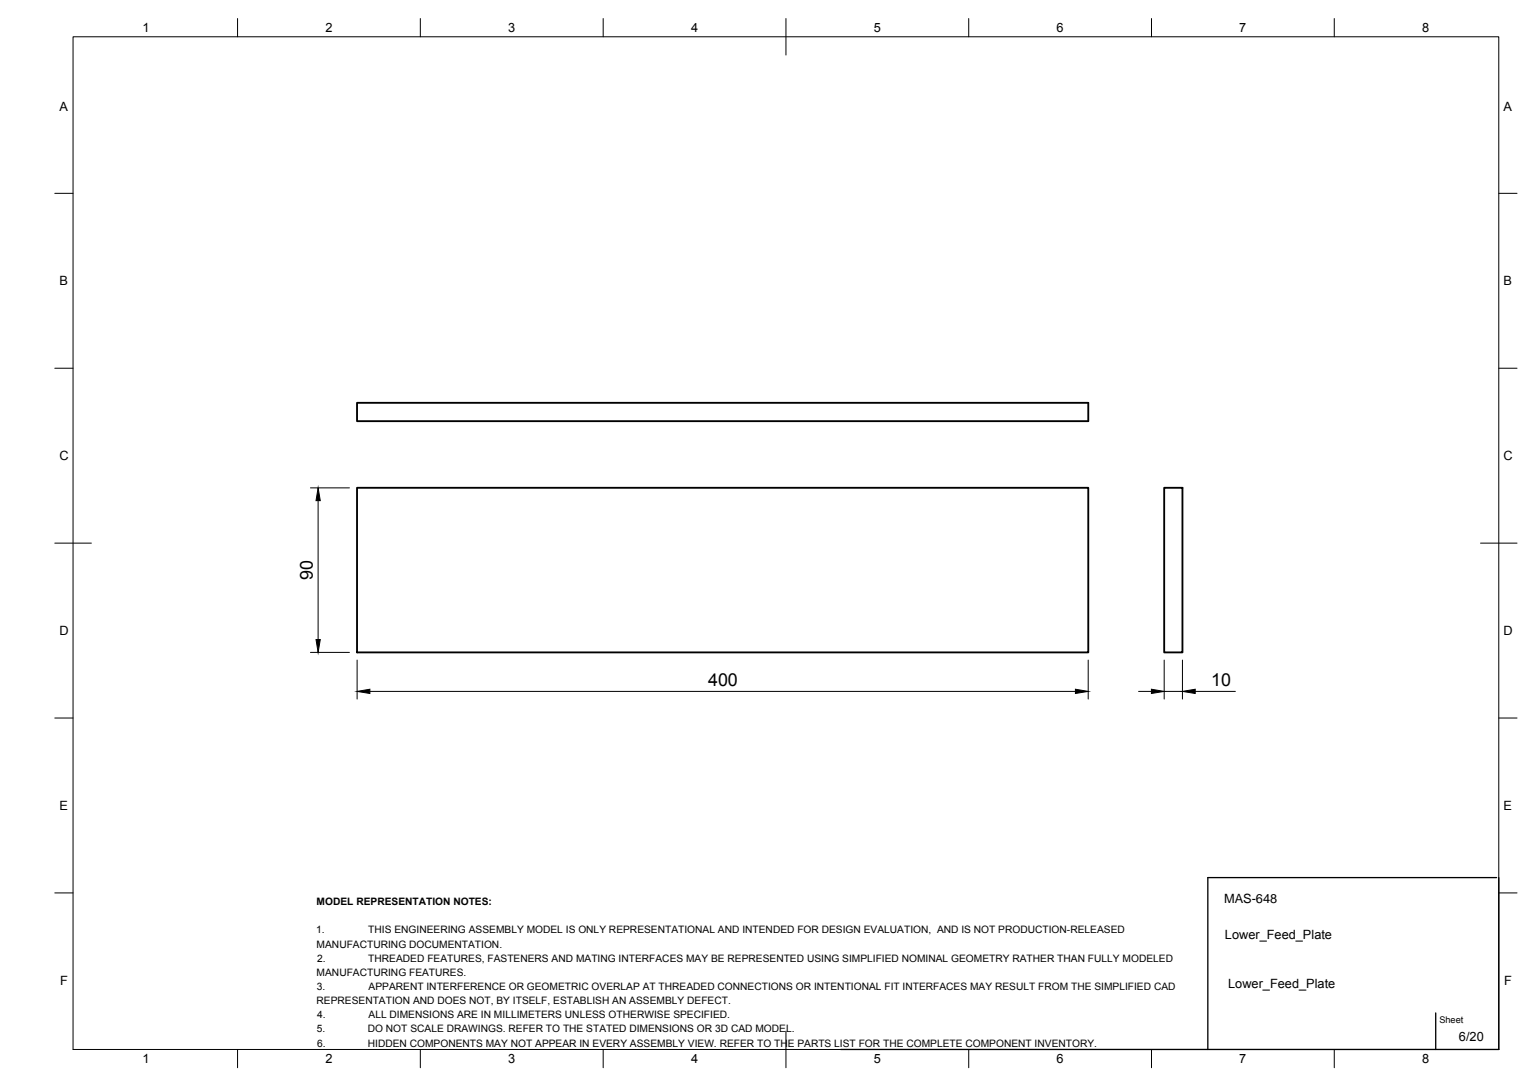
ISO-10303-21;
HEADER;
FILE_DESCRIPTION((''),'2;1');
FILE_NAME('Lower_Feed_Plate.step','2026-10-09T12:47:58-07:00',(''),(''),'','','');
FILE_SCHEMA (('AUTOMOTIVE_DESIGN { 1 0 10303 214 3 1 1 }'));
ENDSEC;
DATA;
#10=MECHANICAL_DESIGN_GEOMETRIC_PRESENTATION_REPRESENTATION('',(#310),#3475);
#286=SHAPE_REPRESENTATION_RELATIONSHIP('SRR','None',#3540,#298) ;
#298=ADVANCED_BREP_SHAPE_REPRESENTATION('',(#322),#3460) ;
#310=STYLED_ITEM('',(#3628),#322) ;
#322=MANIFOLD_SOLID_BREP('Body1',#1824) ;
#334=FACE_OUTER_BOUND('',#448,.T.) ;
#335=FACE_OUTER_BOUND('',#449,.T.) ;
#336=FACE_OUTER_BOUND('',#450,.T.) ;
#337=FACE_OUTER_BOUND('',#451,.T.) ;
#338=FACE_OUTER_BOUND('',#452,.T.) ;
#339=FACE_OUTER_BOUND('',#453,.T.) ;
#448=EDGE_LOOP('',(#1194,#1195,#1196,#1197)) ;
#449=EDGE_LOOP('',(#1198,#1199,#1200,#1201)) ;
#450=EDGE_LOOP('',(#1202,#1203,#1204,#1205)) ;
#451=EDGE_LOOP('',(#1206,#1207,#1208,#1209)) ;
#452=EDGE_LOOP('',(#1210,#1211,#1212,#1213)) ;
#453=EDGE_LOOP('',(#1214,#1215,#1216,#1217)) ;
#587=LINE('',#2829,#706) ;
#588=LINE('',#2831,#707) ;
#589=LINE('',#2833,#708) ;
#590=LINE('',#2834,#709) ;
#591=LINE('',#2837,#710) ;
#592=LINE('',#2839,#711) ;
#593=LINE('',#2840,#712) ;
#594=LINE('',#2843,#713) ;
#595=LINE('',#2845,#714) ;
#596=LINE('',#2846,#715) ;
#597=LINE('',#2848,#716) ;
#598=LINE('',#2849,#717) ;
#706=VECTOR('',#2222,1000.) ;
#707=VECTOR('',#2223,1000.) ;
#708=VECTOR('',#2224,1000.) ;
#709=VECTOR('',#2225,1000.) ;
#710=VECTOR('',#2228,1000.) ;
#711=VECTOR('',#2229,1000.) ;
#712=VECTOR('',#2230,1000.) ;
#713=VECTOR('',#2233,1000.) ;
#714=VECTOR('',#2234,1000.) ;
#715=VECTOR('',#2235,1000.) ;
#716=VECTOR('',#2238,1000.) ;
#717=VECTOR('',#2239,1000.) ;
#825=VERTEX_POINT('',#2827) ;
#826=VERTEX_POINT('',#2828) ;
#827=VERTEX_POINT('',#2830) ;
#828=VERTEX_POINT('',#2832) ;
#829=VERTEX_POINT('',#2836) ;
#830=VERTEX_POINT('',#2838) ;
#831=VERTEX_POINT('',#2842) ;
#832=VERTEX_POINT('',#2844) ;
#969=EDGE_CURVE('',#825,#826,#587,.T.) ;
#970=EDGE_CURVE('',#827,#825,#588,.T.) ;
#971=EDGE_CURVE('',#827,#828,#589,.T.) ;
#972=EDGE_CURVE('',#828,#826,#590,.T.) ;
#973=EDGE_CURVE('',#829,#825,#591,.T.) ;
#974=EDGE_CURVE('',#830,#829,#592,.T.) ;
#975=EDGE_CURVE('',#830,#827,#593,.T.) ;
#976=EDGE_CURVE('',#831,#829,#594,.T.) ;
#977=EDGE_CURVE('',#832,#831,#595,.T.) ;
#978=EDGE_CURVE('',#832,#830,#596,.T.) ;
#979=EDGE_CURVE('',#826,#831,#597,.T.) ;
#980=EDGE_CURVE('',#828,#832,#598,.T.) ;
#1194=ORIENTED_EDGE('',*,*,#969,.F.) ;
#1195=ORIENTED_EDGE('',*,*,#970,.F.) ;
#1196=ORIENTED_EDGE('',*,*,#971,.T.) ;
#1197=ORIENTED_EDGE('',*,*,#972,.T.) ;
#1198=ORIENTED_EDGE('',*,*,#973,.F.) ;
#1199=ORIENTED_EDGE('',*,*,#974,.F.) ;
#1200=ORIENTED_EDGE('',*,*,#975,.T.) ;
#1201=ORIENTED_EDGE('',*,*,#970,.T.) ;
#1202=ORIENTED_EDGE('',*,*,#976,.F.) ;
#1203=ORIENTED_EDGE('',*,*,#977,.F.) ;
#1204=ORIENTED_EDGE('',*,*,#978,.T.) ;
#1205=ORIENTED_EDGE('',*,*,#974,.T.) ;
#1206=ORIENTED_EDGE('',*,*,#979,.F.) ;
#1207=ORIENTED_EDGE('',*,*,#972,.F.) ;
#1208=ORIENTED_EDGE('',*,*,#980,.T.) ;
#1209=ORIENTED_EDGE('',*,*,#977,.T.) ;
#1210=ORIENTED_EDGE('',*,*,#971,.F.) ;
#1211=ORIENTED_EDGE('',*,*,#975,.F.) ;
#1212=ORIENTED_EDGE('',*,*,#978,.F.) ;
#1213=ORIENTED_EDGE('',*,*,#980,.F.) ;
#1214=ORIENTED_EDGE('',*,*,#969,.T.) ;
#1215=ORIENTED_EDGE('',*,*,#979,.T.) ;
#1216=ORIENTED_EDGE('',*,*,#976,.T.) ;
#1217=ORIENTED_EDGE('',*,*,#973,.T.) ;
#1644=PLANE('',#1972) ;
#1645=PLANE('',#1973) ;
#1646=PLANE('',#1974) ;
#1647=PLANE('',#1975) ;
#1648=PLANE('',#1976) ;
#1649=PLANE('',#1977) ;
#1710=ADVANCED_FACE('',(#334),#1644,.T.) ;
#1711=ADVANCED_FACE('',(#335),#1645,.T.) ;
#1712=ADVANCED_FACE('',(#336),#1646,.T.) ;
#1713=ADVANCED_FACE('',(#337),#1647,.T.) ;
#1714=ADVANCED_FACE('',(#338),#1648,.F.) ;
#1715=ADVANCED_FACE('',(#339),#1649,.T.) ;
#1824=CLOSED_SHELL('',(#1710,#1711,#1712,#1713,#1714,#1715)) ;
#1971=AXIS2_PLACEMENT_3D('',#2825,#2218,#2219) ;
#1972=AXIS2_PLACEMENT_3D('',#2826,#2220,#2221) ;
#1973=AXIS2_PLACEMENT_3D('',#2835,#2226,#2227) ;
#1974=AXIS2_PLACEMENT_3D('',#2841,#2231,#2232) ;
#1975=AXIS2_PLACEMENT_3D('',#2847,#2236,#2237) ;
#1976=AXIS2_PLACEMENT_3D('',#2850,#2240,#2241) ;
#1977=AXIS2_PLACEMENT_3D('',#2851,#2242,#2243) ;
#2218=DIRECTION('axis',(0.,0.,1.)) ;
#2219=DIRECTION('refdir',(1.,0.,0.)) ;
#2220=DIRECTION('center_axis',(-1.,0.,0.)) ;
#2221=DIRECTION('ref_axis',(0.,0.,1.)) ;
#2222=DIRECTION('',(0.,-1.,0.)) ;
#2223=DIRECTION('',(0.,0.,1.)) ;
#2224=DIRECTION('',(0.,-1.,0.)) ;
#2225=DIRECTION('',(0.,0.,1.)) ;
#2226=DIRECTION('center_axis',(-1.21430643318376E-16,1.,0.)) ;
#2227=DIRECTION('ref_axis',(-1.,-1.21430643318376E-16,0.)) ;
#2228=DIRECTION('',(-1.,-1.21430643318376E-16,0.)) ;
#2229=DIRECTION('',(0.,0.,1.)) ;
#2230=DIRECTION('',(-1.,-1.21430643318376E-16,0.)) ;
#2231=DIRECTION('center_axis',(1.,0.,0.)) ;
#2232=DIRECTION('ref_axis',(0.,0.,-1.)) ;
#2233=DIRECTION('',(0.,1.,0.)) ;
#2234=DIRECTION('',(0.,0.,1.)) ;
#2235=DIRECTION('',(0.,1.,0.)) ;
#2236=DIRECTION('center_axis',(1.21430643318376E-16,-1.,0.)) ;
#2237=DIRECTION('ref_axis',(1.,1.21430643318376E-16,0.)) ;
#2238=DIRECTION('',(1.,1.21430643318376E-16,0.)) ;
#2239=DIRECTION('',(1.,1.21430643318376E-16,0.)) ;
#2240=DIRECTION('center_axis',(0.,0.,1.)) ;
#2241=DIRECTION('ref_axis',(1.,0.,0.)) ;
#2242=DIRECTION('center_axis',(0.,0.,1.)) ;
#2243=DIRECTION('ref_axis',(1.,0.,0.)) ;
#2825=CARTESIAN_POINT('',(0.,0.,0.)) ;
#2826=CARTESIAN_POINT('Origin',(-200.,-45.,-10.)) ;
#2827=CARTESIAN_POINT('',(-200.,45.,0.)) ;
#2828=CARTESIAN_POINT('',(-200.,-45.,0.)) ;
#2829=CARTESIAN_POINT('',(-200.,-45.,0.)) ;
#2830=CARTESIAN_POINT('',(-200.,45.,-10.)) ;
#2831=CARTESIAN_POINT('',(-200.,45.,-10.)) ;
#2832=CARTESIAN_POINT('',(-200.,-45.,-10.)) ;
#2833=CARTESIAN_POINT('',(-200.,-45.,-10.)) ;
#2834=CARTESIAN_POINT('',(-200.,-45.,-10.)) ;
#2835=CARTESIAN_POINT('Origin',(200.,45.,-10.)) ;
#2836=CARTESIAN_POINT('',(200.,45.,0.)) ;
#2837=CARTESIAN_POINT('',(200.,45.,0.)) ;
#2838=CARTESIAN_POINT('',(200.,45.,-10.)) ;
#2839=CARTESIAN_POINT('',(200.,45.,-10.)) ;
#2840=CARTESIAN_POINT('',(200.,45.,-10.)) ;
#2841=CARTESIAN_POINT('Origin',(200.,-45.,-10.)) ;
#2842=CARTESIAN_POINT('',(200.,-45.,0.)) ;
#2843=CARTESIAN_POINT('',(200.,-45.,0.)) ;
#2844=CARTESIAN_POINT('',(200.,-45.,-10.)) ;
#2845=CARTESIAN_POINT('',(200.,-45.,-10.)) ;
#2846=CARTESIAN_POINT('',(200.,-45.,-10.)) ;
#2847=CARTESIAN_POINT('Origin',(200.,-45.,-10.)) ;
#2848=CARTESIAN_POINT('',(200.,-45.,0.)) ;
#2849=CARTESIAN_POINT('',(200.,-45.,-10.)) ;
#2850=CARTESIAN_POINT('Origin',(0.,0.,-10.)) ;
#2851=CARTESIAN_POINT('Origin',(0.,0.,0.)) ;
#3442=UNCERTAINTY_MEASURE_WITH_UNIT(LENGTH_MEASURE(0.01),#3476,
'DISTANCE_ACCURACY_VALUE',
'Maximum model space distance between geometric entities at asserted c
onnectivities') ;
#3457=UNCERTAINTY_MEASURE_WITH_UNIT(LENGTH_MEASURE(0.01),#3476,
'DISTANCE_ACCURACY_VALUE',
'Maximum model space distance between geometric entities at asserted c
onnectivities') ;
#3460=(
GEOMETRIC_REPRESENTATION_CONTEXT(3)
GLOBAL_UNCERTAINTY_ASSIGNED_CONTEXT((#3442))
GLOBAL_UNIT_ASSIGNED_CONTEXT((#3476,#3478,#3479))
REPRESENTATION_CONTEXT('','3D')
) ;
#3475=(
GEOMETRIC_REPRESENTATION_CONTEXT(3)
GLOBAL_UNCERTAINTY_ASSIGNED_CONTEXT((#3457))
GLOBAL_UNIT_ASSIGNED_CONTEXT((#3476,#3478,#3479))
REPRESENTATION_CONTEXT('','3D')
) ;
#3476=(
LENGTH_UNIT()
NAMED_UNIT(*)
SI_UNIT(.MILLI.,.METRE.)
) ;
#3478=(
NAMED_UNIT(*)
PLANE_ANGLE_UNIT()
SI_UNIT($,.RADIAN.)
) ;
#3479=(
NAMED_UNIT(*)
SI_UNIT($,.STERADIAN.)
SOLID_ANGLE_UNIT()
) ;
#3482=SHAPE_DEFINITION_REPRESENTATION(#3499,#3540) ;
#3499=PRODUCT_DEFINITION_SHAPE('',$,#3558) ;
#3540=SHAPE_REPRESENTATION('',(#1971),#3460) ;
#3555=PRODUCT_DEFINITION_CONTEXT('part definition',#3608,'design') ;
#3558=PRODUCT_DEFINITION('Lower_Feed_Plate','Lower_Feed_Plate',#3575,#3555) ;
#3575=PRODUCT_DEFINITION_FORMATION('',$,#3612) ;
#3608=APPLICATION_CONTEXT(
'Core Data for Automotive Mechanical Design Process') ;
#3609=PRODUCT_CONTEXT('part definition',#3608,'mechanical') ;
#3612=PRODUCT('Lower_Feed_Plate',
'Lower_Feed_Plate',$,(#3609)) ;
#3628=PRESENTATION_STYLE_ASSIGNMENT((#3630)) ;
#3630=SURFACE_STYLE_USAGE(.BOTH.,#3632) ;
#3632=SURFACE_SIDE_STYLE('',(#3634)) ;
#3634=SURFACE_STYLE_FILL_AREA(#3636) ;
#3636=FILL_AREA_STYLE('Opaque(202,209,238)',(#3638)) ;
#3638=FILL_AREA_STYLE_COLOUR('Opaque(202,209,238)',#3640) ;
#3640=COLOUR_RGB('Opaque(202,209,238)', 0.09019608, 0.27058824, 0.51372549) ;
ENDSEC;
END-ISO-10303-21;
